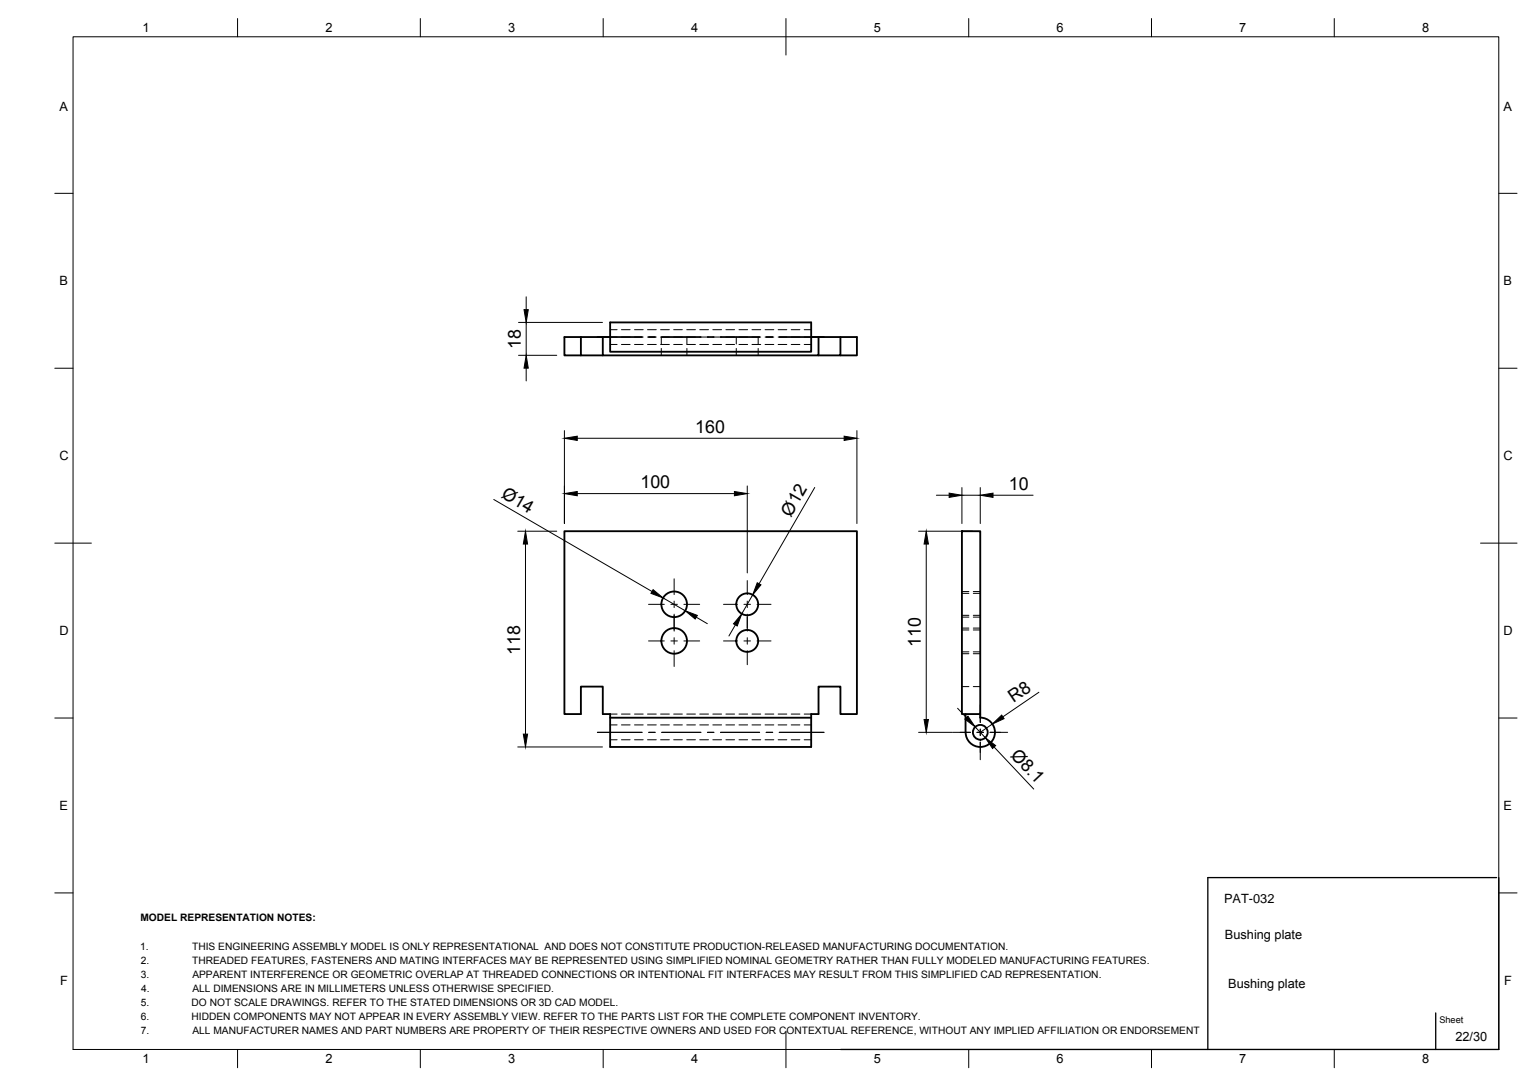
ISO-10303-21;
HEADER;
/* Generated by software containing ST-Developer
 * from STEP Tools, Inc. (www.steptools.com) 
 */

FILE_DESCRIPTION(
/* description */ ('Drill jig with bushing plate'),
/* implementation_level */ '2;1');

FILE_NAME(
/* name */ 'Bushing plate.step',
/* time_stamp */ '2026-10-27T10:51:08-07:00',
/* author */ (''),
/* organization */ (''),
/* preprocessor_version */ 'ST-DEVELOPER v20.2',
/* originating_system */ 'Autodesk Translation Framework v15.17.0.0',
/* authorisation */ '');

FILE_SCHEMA (('AUTOMOTIVE_DESIGN { 1 0 10303 214 3 1 1 }'));
ENDSEC;

DATA;
#10=MECHANICAL_DESIGN_GEOMETRIC_PRESENTATION_REPRESENTATION('',(#240),#6638);
#192=SHAPE_REPRESENTATION_RELATIONSHIP('SRR','None',#6757,#216);
#216=ADVANCED_BREP_SHAPE_REPRESENTATION('',(#262),#6630);
#240=STYLED_ITEM('',(#6957),#262);
#262=MANIFOLD_SOLID_BREP('Body1',#3609);
#345=FACE_BOUND('',#951,.T.);
#346=FACE_BOUND('',#954,.T.);
#347=FACE_BOUND('',#962,.T.);
#348=FACE_BOUND('',#963,.T.);
#349=FACE_BOUND('',#964,.T.);
#350=FACE_BOUND('',#965,.T.);
#351=FACE_BOUND('',#975,.T.);
#352=FACE_BOUND('',#976,.T.);
#353=FACE_BOUND('',#977,.T.);
#354=FACE_BOUND('',#978,.T.);
#464=PLANE('',#4221);
#465=PLANE('',#4224);
#466=PLANE('',#4225);
#467=PLANE('',#4230);
#468=PLANE('',#4231);
#469=PLANE('',#4232);
#470=PLANE('',#4233);
#471=PLANE('',#4234);
#472=PLANE('',#4235);
#473=PLANE('',#4236);
#474=PLANE('',#4237);
#475=PLANE('',#4238);
#476=PLANE('',#4239);
#477=PLANE('',#4240);
#478=PLANE('',#4241);
#479=PLANE('',#4242);
#480=PLANE('',#4243);
#656=FACE_OUTER_BOUND('',#946,.T.);
#657=FACE_OUTER_BOUND('',#947,.T.);
#658=FACE_OUTER_BOUND('',#948,.T.);
#659=FACE_OUTER_BOUND('',#949,.T.);
#660=FACE_OUTER_BOUND('',#950,.T.);
#661=FACE_OUTER_BOUND('',#952,.T.);
#662=FACE_OUTER_BOUND('',#953,.T.);
#663=FACE_OUTER_BOUND('',#955,.T.);
#664=FACE_OUTER_BOUND('',#956,.T.);
#665=FACE_OUTER_BOUND('',#957,.T.);
#666=FACE_OUTER_BOUND('',#958,.T.);
#667=FACE_OUTER_BOUND('',#959,.T.);
#668=FACE_OUTER_BOUND('',#960,.T.);
#669=FACE_OUTER_BOUND('',#961,.T.);
#670=FACE_OUTER_BOUND('',#966,.T.);
#671=FACE_OUTER_BOUND('',#967,.T.);
#672=FACE_OUTER_BOUND('',#968,.T.);
#673=FACE_OUTER_BOUND('',#969,.T.);
#674=FACE_OUTER_BOUND('',#970,.T.);
#675=FACE_OUTER_BOUND('',#971,.T.);
#676=FACE_OUTER_BOUND('',#972,.T.);
#677=FACE_OUTER_BOUND('',#973,.T.);
#678=FACE_OUTER_BOUND('',#974,.T.);
#946=EDGE_LOOP('',(#3059,#3060,#3061,#3062));
#947=EDGE_LOOP('',(#3063,#3064,#3065,#3066));
#948=EDGE_LOOP('',(#3067,#3068,#3069,#3070));
#949=EDGE_LOOP('',(#3071,#3072,#3073,#3074));
#950=EDGE_LOOP('',(#3075,#3076,#3077,#3078));
#951=EDGE_LOOP('',(#3079));
#952=EDGE_LOOP('',(#3080,#3081,#3082,#3083));
#953=EDGE_LOOP('',(#3084,#3085,#3086,#3087));
#954=EDGE_LOOP('',(#3088));
#955=EDGE_LOOP('',(#3089,#3090,#3091,#3092));
#956=EDGE_LOOP('',(#3093,#3094,#3095,#3096));
#957=EDGE_LOOP('',(#3097,#3098,#3099,#3100,#3101,#3102,#3103,#3104));
#958=EDGE_LOOP('',(#3105,#3106,#3107,#3108));
#959=EDGE_LOOP('',(#3109,#3110,#3111,#3112));
#960=EDGE_LOOP('',(#3113,#3114,#3115,#3116));
#961=EDGE_LOOP('',(#3117,#3118,#3119,#3120,#3121,#3122,#3123,#3124,#3125,
#3126,#3127,#3128,#3129,#3130,#3131,#3132));
#962=EDGE_LOOP('',(#3133));
#963=EDGE_LOOP('',(#3134));
#964=EDGE_LOOP('',(#3135));
#965=EDGE_LOOP('',(#3136));
#966=EDGE_LOOP('',(#3137,#3138,#3139,#3140));
#967=EDGE_LOOP('',(#3141,#3142,#3143,#3144));
#968=EDGE_LOOP('',(#3145,#3146,#3147,#3148));
#969=EDGE_LOOP('',(#3149,#3150,#3151,#3152));
#970=EDGE_LOOP('',(#3153,#3154,#3155,#3156));
#971=EDGE_LOOP('',(#3157,#3158,#3159,#3160));
#972=EDGE_LOOP('',(#3161,#3162,#3163,#3164));
#973=EDGE_LOOP('',(#3165,#3166,#3167,#3168));
#974=EDGE_LOOP('',(#3169,#3170,#3171,#3172,#3173,#3174,#3175,#3176,#3177,
#3178,#3179,#3180));
#975=EDGE_LOOP('',(#3181));
#976=EDGE_LOOP('',(#3182));
#977=EDGE_LOOP('',(#3183));
#978=EDGE_LOOP('',(#3184));
#1215=LINE('',#6309,#1476);
#1216=LINE('',#6315,#1477);
#1217=LINE('',#6321,#1478);
#1218=LINE('',#6327,#1479);
#1219=LINE('',#6334,#1480);
#1220=LINE('',#6336,#1481);
#1221=LINE('',#6337,#1482);
#1222=LINE('',#6342,#1483);
#1223=LINE('',#6344,#1484);
#1224=LINE('',#6345,#1485);
#1225=LINE('',#6350,#1486);
#1226=LINE('',#6351,#1487);
#1227=LINE('',#6355,#1488);
#1228=LINE('',#6357,#1489);
#1229=LINE('',#6360,#1490);
#1230=LINE('',#6362,#1491);
#1231=LINE('',#6364,#1492);
#1232=LINE('',#6366,#1493);
#1233=LINE('',#6367,#1494);
#1234=LINE('',#6370,#1495);
#1235=LINE('',#6372,#1496);
#1236=LINE('',#6373,#1497);
#1237=LINE('',#6376,#1498);
#1238=LINE('',#6378,#1499);
#1239=LINE('',#6379,#1500);
#1240=LINE('',#6382,#1501);
#1241=LINE('',#6384,#1502);
#1242=LINE('',#6385,#1503);
#1243=LINE('',#6388,#1504);
#1244=LINE('',#6390,#1505);
#1245=LINE('',#6392,#1506);
#1246=LINE('',#6394,#1507);
#1247=LINE('',#6396,#1508);
#1248=LINE('',#6398,#1509);
#1249=LINE('',#6400,#1510);
#1250=LINE('',#6401,#1511);
#1251=LINE('',#6404,#1512);
#1252=LINE('',#6405,#1513);
#1253=LINE('',#6408,#1514);
#1254=LINE('',#6409,#1515);
#1255=LINE('',#6412,#1516);
#1256=LINE('',#6413,#1517);
#1257=LINE('',#6416,#1518);
#1258=LINE('',#6417,#1519);
#1259=LINE('',#6420,#1520);
#1260=LINE('',#6421,#1521);
#1261=LINE('',#6424,#1522);
#1262=LINE('',#6426,#1523);
#1263=LINE('',#6427,#1524);
#1264=LINE('',#6429,#1525);
#1265=LINE('',#6431,#1526);
#1476=VECTOR('',#5174,0.7);
#1477=VECTOR('',#5181,0.7);
#1478=VECTOR('',#5188,0.6);
#1479=VECTOR('',#5195,0.6);
#1480=VECTOR('',#5202,1.);
#1481=VECTOR('',#5203,1.);
#1482=VECTOR('',#5204,1.);
#1483=VECTOR('',#5209,1.);
#1484=VECTOR('',#5210,1.);
#1485=VECTOR('',#5211,1.);
#1486=VECTOR('',#5216,1.);
#1487=VECTOR('',#5217,1.);
#1488=VECTOR('',#5222,0.405);
#1489=VECTOR('',#5225,1.);
#1490=VECTOR('',#5228,1.);
#1491=VECTOR('',#5229,1.);
#1492=VECTOR('',#5230,1.);
#1493=VECTOR('',#5231,1.);
#1494=VECTOR('',#5232,1.);
#1495=VECTOR('',#5235,1.);
#1496=VECTOR('',#5236,1.);
#1497=VECTOR('',#5237,1.);
#1498=VECTOR('',#5240,1.);
#1499=VECTOR('',#5241,1.);
#1500=VECTOR('',#5242,1.);
#1501=VECTOR('',#5245,1.);
#1502=VECTOR('',#5246,1.);
#1503=VECTOR('',#5247,1.);
#1504=VECTOR('',#5250,1.);
#1505=VECTOR('',#5251,1.);
#1506=VECTOR('',#5252,1.);
#1507=VECTOR('',#5253,1.);
#1508=VECTOR('',#5254,1.);
#1509=VECTOR('',#5255,1.);
#1510=VECTOR('',#5256,1.);
#1511=VECTOR('',#5257,1.);
#1512=VECTOR('',#5260,1.);
#1513=VECTOR('',#5261,1.);
#1514=VECTOR('',#5264,1.);
#1515=VECTOR('',#5265,1.);
#1516=VECTOR('',#5268,1.);
#1517=VECTOR('',#5269,1.);
#1518=VECTOR('',#5272,1.);
#1519=VECTOR('',#5273,1.);
#1520=VECTOR('',#5276,1.);
#1521=VECTOR('',#5277,1.);
#1522=VECTOR('',#5280,1.);
#1523=VECTOR('',#5281,1.);
#1524=VECTOR('',#5282,1.);
#1525=VECTOR('',#5285,1.);
#1526=VECTOR('',#5288,1.);
#1676=CIRCLE('',#4210,0.7);
#1677=CIRCLE('',#4211,0.7);
#1678=CIRCLE('',#4213,0.7);
#1679=CIRCLE('',#4214,0.7);
#1680=CIRCLE('',#4216,0.6);
#1681=CIRCLE('',#4217,0.6);
#1682=CIRCLE('',#4219,0.6);
#1683=CIRCLE('',#4220,0.6);
#1684=CIRCLE('',#4222,0.8);
#1685=CIRCLE('',#4223,0.405);
#1686=CIRCLE('',#4226,0.8);
#1687=CIRCLE('',#4227,0.405);
#1926=VERTEX_POINT('',#6306);
#1927=VERTEX_POINT('',#6308);
#1928=VERTEX_POINT('',#6312);
#1929=VERTEX_POINT('',#6314);
#1930=VERTEX_POINT('',#6318);
#1931=VERTEX_POINT('',#6320);
#1932=VERTEX_POINT('',#6324);
#1933=VERTEX_POINT('',#6326);
#1934=VERTEX_POINT('',#6330);
#1935=VERTEX_POINT('',#6331);
#1936=VERTEX_POINT('',#6333);
#1937=VERTEX_POINT('',#6335);
#1938=VERTEX_POINT('',#6338);
#1939=VERTEX_POINT('',#6341);
#1940=VERTEX_POINT('',#6343);
#1941=VERTEX_POINT('',#6347);
#1942=VERTEX_POINT('',#6349);
#1943=VERTEX_POINT('',#6352);
#1944=VERTEX_POINT('',#6359);
#1945=VERTEX_POINT('',#6361);
#1946=VERTEX_POINT('',#6363);
#1947=VERTEX_POINT('',#6365);
#1948=VERTEX_POINT('',#6369);
#1949=VERTEX_POINT('',#6371);
#1950=VERTEX_POINT('',#6375);
#1951=VERTEX_POINT('',#6377);
#1952=VERTEX_POINT('',#6381);
#1953=VERTEX_POINT('',#6383);
#1954=VERTEX_POINT('',#6387);
#1955=VERTEX_POINT('',#6389);
#1956=VERTEX_POINT('',#6391);
#1957=VERTEX_POINT('',#6393);
#1958=VERTEX_POINT('',#6395);
#1959=VERTEX_POINT('',#6397);
#1960=VERTEX_POINT('',#6399);
#1961=VERTEX_POINT('',#6403);
#1962=VERTEX_POINT('',#6407);
#1963=VERTEX_POINT('',#6411);
#1964=VERTEX_POINT('',#6415);
#1965=VERTEX_POINT('',#6419);
#1966=VERTEX_POINT('',#6423);
#1967=VERTEX_POINT('',#6425);
#2317=EDGE_CURVE('',#1926,#1926,#1676,.T.);
#2318=EDGE_CURVE('',#1926,#1927,#1215,.T.);
#2319=EDGE_CURVE('',#1927,#1927,#1677,.T.);
#2320=EDGE_CURVE('',#1928,#1928,#1678,.T.);
#2321=EDGE_CURVE('',#1928,#1929,#1216,.T.);
#2322=EDGE_CURVE('',#1929,#1929,#1679,.T.);
#2323=EDGE_CURVE('',#1930,#1930,#1680,.T.);
#2324=EDGE_CURVE('',#1930,#1931,#1217,.T.);
#2325=EDGE_CURVE('',#1931,#1931,#1681,.T.);
#2326=EDGE_CURVE('',#1932,#1932,#1682,.T.);
#2327=EDGE_CURVE('',#1932,#1933,#1218,.T.);
#2328=EDGE_CURVE('',#1933,#1933,#1683,.T.);
#2329=EDGE_CURVE('',#1934,#1935,#1684,.T.);
#2330=EDGE_CURVE('',#1936,#1934,#1219,.T.);
#2331=EDGE_CURVE('',#1937,#1936,#1220,.T.);
#2332=EDGE_CURVE('',#1935,#1937,#1221,.T.);
#2333=EDGE_CURVE('',#1938,#1938,#1685,.T.);
#2334=EDGE_CURVE('',#1936,#1939,#1222,.T.);
#2335=EDGE_CURVE('',#1934,#1940,#1223,.T.);
#2336=EDGE_CURVE('',#1939,#1940,#1224,.T.);
#2337=EDGE_CURVE('',#1940,#1941,#1686,.T.);
#2338=EDGE_CURVE('',#1941,#1942,#1225,.T.);
#2339=EDGE_CURVE('',#1939,#1942,#1226,.T.);
#2340=EDGE_CURVE('',#1943,#1943,#1687,.T.);
#2341=EDGE_CURVE('',#1943,#1938,#1227,.T.);
#2342=EDGE_CURVE('',#1935,#1941,#1228,.T.);
#2343=EDGE_CURVE('',#1942,#1944,#1229,.T.);
#2344=EDGE_CURVE('',#1944,#1945,#1230,.T.);
#2345=EDGE_CURVE('',#1946,#1945,#1231,.T.);
#2346=EDGE_CURVE('',#1946,#1947,#1232,.T.);
#2347=EDGE_CURVE('',#1947,#1937,#1233,.T.);
#2348=EDGE_CURVE('',#1948,#1944,#1234,.T.);
#2349=EDGE_CURVE('',#1948,#1949,#1235,.T.);
#2350=EDGE_CURVE('',#1945,#1949,#1236,.T.);
#2351=EDGE_CURVE('',#1950,#1948,#1237,.T.);
#2352=EDGE_CURVE('',#1950,#1951,#1238,.T.);
#2353=EDGE_CURVE('',#1949,#1951,#1239,.T.);
#2354=EDGE_CURVE('',#1952,#1950,#1240,.T.);
#2355=EDGE_CURVE('',#1953,#1952,#1241,.T.);
#2356=EDGE_CURVE('',#1951,#1953,#1242,.T.);
#2357=EDGE_CURVE('',#1947,#1954,#1243,.T.);
#2358=EDGE_CURVE('',#1954,#1955,#1244,.T.);
#2359=EDGE_CURVE('',#1955,#1956,#1245,.T.);
#2360=EDGE_CURVE('',#1957,#1956,#1246,.T.);
#2361=EDGE_CURVE('',#1958,#1957,#1247,.T.);
#2362=EDGE_CURVE('',#1959,#1958,#1248,.T.);
#2363=EDGE_CURVE('',#1960,#1959,#1249,.T.);
#2364=EDGE_CURVE('',#1952,#1960,#1250,.T.);
#2365=EDGE_CURVE('',#1961,#1946,#1251,.T.);
#2366=EDGE_CURVE('',#1954,#1961,#1252,.T.);
#2367=EDGE_CURVE('',#1962,#1961,#1253,.T.);
#2368=EDGE_CURVE('',#1955,#1962,#1254,.T.);
#2369=EDGE_CURVE('',#1963,#1962,#1255,.T.);
#2370=EDGE_CURVE('',#1956,#1963,#1256,.T.);
#2371=EDGE_CURVE('',#1964,#1963,#1257,.T.);
#2372=EDGE_CURVE('',#1957,#1964,#1258,.T.);
#2373=EDGE_CURVE('',#1960,#1965,#1259,.T.);
#2374=EDGE_CURVE('',#1953,#1965,#1260,.T.);
#2375=EDGE_CURVE('',#1958,#1966,#1261,.T.);
#2376=EDGE_CURVE('',#1967,#1966,#1262,.T.);
#2377=EDGE_CURVE('',#1959,#1967,#1263,.T.);
#2378=EDGE_CURVE('',#1965,#1967,#1264,.T.);
#2379=EDGE_CURVE('',#1966,#1964,#1265,.T.);
#3059=ORIENTED_EDGE('',*,*,#2317,.F.);
#3060=ORIENTED_EDGE('',*,*,#2318,.T.);
#3061=ORIENTED_EDGE('',*,*,#2319,.F.);
#3062=ORIENTED_EDGE('',*,*,#2318,.F.);
#3063=ORIENTED_EDGE('',*,*,#2320,.F.);
#3064=ORIENTED_EDGE('',*,*,#2321,.T.);
#3065=ORIENTED_EDGE('',*,*,#2322,.F.);
#3066=ORIENTED_EDGE('',*,*,#2321,.F.);
#3067=ORIENTED_EDGE('',*,*,#2323,.F.);
#3068=ORIENTED_EDGE('',*,*,#2324,.T.);
#3069=ORIENTED_EDGE('',*,*,#2325,.F.);
#3070=ORIENTED_EDGE('',*,*,#2324,.F.);
#3071=ORIENTED_EDGE('',*,*,#2326,.F.);
#3072=ORIENTED_EDGE('',*,*,#2327,.T.);
#3073=ORIENTED_EDGE('',*,*,#2328,.F.);
#3074=ORIENTED_EDGE('',*,*,#2327,.F.);
#3075=ORIENTED_EDGE('',*,*,#2329,.F.);
#3076=ORIENTED_EDGE('',*,*,#2330,.F.);
#3077=ORIENTED_EDGE('',*,*,#2331,.F.);
#3078=ORIENTED_EDGE('',*,*,#2332,.F.);
#3079=ORIENTED_EDGE('',*,*,#2333,.F.);
#3080=ORIENTED_EDGE('',*,*,#2334,.F.);
#3081=ORIENTED_EDGE('',*,*,#2330,.T.);
#3082=ORIENTED_EDGE('',*,*,#2335,.T.);
#3083=ORIENTED_EDGE('',*,*,#2336,.F.);
#3084=ORIENTED_EDGE('',*,*,#2337,.T.);
#3085=ORIENTED_EDGE('',*,*,#2338,.T.);
#3086=ORIENTED_EDGE('',*,*,#2339,.F.);
#3087=ORIENTED_EDGE('',*,*,#2336,.T.);
#3088=ORIENTED_EDGE('',*,*,#2340,.T.);
#3089=ORIENTED_EDGE('',*,*,#2340,.F.);
#3090=ORIENTED_EDGE('',*,*,#2341,.T.);
#3091=ORIENTED_EDGE('',*,*,#2333,.T.);
#3092=ORIENTED_EDGE('',*,*,#2341,.F.);
#3093=ORIENTED_EDGE('',*,*,#2342,.T.);
#3094=ORIENTED_EDGE('',*,*,#2337,.F.);
#3095=ORIENTED_EDGE('',*,*,#2335,.F.);
#3096=ORIENTED_EDGE('',*,*,#2329,.T.);
#3097=ORIENTED_EDGE('',*,*,#2331,.T.);
#3098=ORIENTED_EDGE('',*,*,#2334,.T.);
#3099=ORIENTED_EDGE('',*,*,#2339,.T.);
#3100=ORIENTED_EDGE('',*,*,#2343,.T.);
#3101=ORIENTED_EDGE('',*,*,#2344,.T.);
#3102=ORIENTED_EDGE('',*,*,#2345,.F.);
#3103=ORIENTED_EDGE('',*,*,#2346,.T.);
#3104=ORIENTED_EDGE('',*,*,#2347,.T.);
#3105=ORIENTED_EDGE('',*,*,#2348,.F.);
#3106=ORIENTED_EDGE('',*,*,#2349,.T.);
#3107=ORIENTED_EDGE('',*,*,#2350,.F.);
#3108=ORIENTED_EDGE('',*,*,#2344,.F.);
#3109=ORIENTED_EDGE('',*,*,#2351,.F.);
#3110=ORIENTED_EDGE('',*,*,#2352,.T.);
#3111=ORIENTED_EDGE('',*,*,#2353,.F.);
#3112=ORIENTED_EDGE('',*,*,#2349,.F.);
#3113=ORIENTED_EDGE('',*,*,#2354,.F.);
#3114=ORIENTED_EDGE('',*,*,#2355,.F.);
#3115=ORIENTED_EDGE('',*,*,#2356,.F.);
#3116=ORIENTED_EDGE('',*,*,#2352,.F.);
#3117=ORIENTED_EDGE('',*,*,#2347,.F.);
#3118=ORIENTED_EDGE('',*,*,#2357,.T.);
#3119=ORIENTED_EDGE('',*,*,#2358,.T.);
#3120=ORIENTED_EDGE('',*,*,#2359,.T.);
#3121=ORIENTED_EDGE('',*,*,#2360,.F.);
#3122=ORIENTED_EDGE('',*,*,#2361,.F.);
#3123=ORIENTED_EDGE('',*,*,#2362,.F.);
#3124=ORIENTED_EDGE('',*,*,#2363,.F.);
#3125=ORIENTED_EDGE('',*,*,#2364,.F.);
#3126=ORIENTED_EDGE('',*,*,#2354,.T.);
#3127=ORIENTED_EDGE('',*,*,#2351,.T.);
#3128=ORIENTED_EDGE('',*,*,#2348,.T.);
#3129=ORIENTED_EDGE('',*,*,#2343,.F.);
#3130=ORIENTED_EDGE('',*,*,#2338,.F.);
#3131=ORIENTED_EDGE('',*,*,#2342,.F.);
#3132=ORIENTED_EDGE('',*,*,#2332,.T.);
#3133=ORIENTED_EDGE('',*,*,#2317,.T.);
#3134=ORIENTED_EDGE('',*,*,#2320,.T.);
#3135=ORIENTED_EDGE('',*,*,#2323,.T.);
#3136=ORIENTED_EDGE('',*,*,#2326,.T.);
#3137=ORIENTED_EDGE('',*,*,#2365,.F.);
#3138=ORIENTED_EDGE('',*,*,#2366,.F.);
#3139=ORIENTED_EDGE('',*,*,#2357,.F.);
#3140=ORIENTED_EDGE('',*,*,#2346,.F.);
#3141=ORIENTED_EDGE('',*,*,#2367,.F.);
#3142=ORIENTED_EDGE('',*,*,#2368,.F.);
#3143=ORIENTED_EDGE('',*,*,#2358,.F.);
#3144=ORIENTED_EDGE('',*,*,#2366,.T.);
#3145=ORIENTED_EDGE('',*,*,#2369,.F.);
#3146=ORIENTED_EDGE('',*,*,#2370,.F.);
#3147=ORIENTED_EDGE('',*,*,#2359,.F.);
#3148=ORIENTED_EDGE('',*,*,#2368,.T.);
#3149=ORIENTED_EDGE('',*,*,#2370,.T.);
#3150=ORIENTED_EDGE('',*,*,#2371,.F.);
#3151=ORIENTED_EDGE('',*,*,#2372,.F.);
#3152=ORIENTED_EDGE('',*,*,#2360,.T.);
#3153=ORIENTED_EDGE('',*,*,#2355,.T.);
#3154=ORIENTED_EDGE('',*,*,#2364,.T.);
#3155=ORIENTED_EDGE('',*,*,#2373,.T.);
#3156=ORIENTED_EDGE('',*,*,#2374,.F.);
#3157=ORIENTED_EDGE('',*,*,#2362,.T.);
#3158=ORIENTED_EDGE('',*,*,#2375,.T.);
#3159=ORIENTED_EDGE('',*,*,#2376,.F.);
#3160=ORIENTED_EDGE('',*,*,#2377,.F.);
#3161=ORIENTED_EDGE('',*,*,#2363,.T.);
#3162=ORIENTED_EDGE('',*,*,#2377,.T.);
#3163=ORIENTED_EDGE('',*,*,#2378,.F.);
#3164=ORIENTED_EDGE('',*,*,#2373,.F.);
#3165=ORIENTED_EDGE('',*,*,#2361,.T.);
#3166=ORIENTED_EDGE('',*,*,#2372,.T.);
#3167=ORIENTED_EDGE('',*,*,#2379,.F.);
#3168=ORIENTED_EDGE('',*,*,#2375,.F.);
#3169=ORIENTED_EDGE('',*,*,#2356,.T.);
#3170=ORIENTED_EDGE('',*,*,#2374,.T.);
#3171=ORIENTED_EDGE('',*,*,#2378,.T.);
#3172=ORIENTED_EDGE('',*,*,#2376,.T.);
#3173=ORIENTED_EDGE('',*,*,#2379,.T.);
#3174=ORIENTED_EDGE('',*,*,#2371,.T.);
#3175=ORIENTED_EDGE('',*,*,#2369,.T.);
#3176=ORIENTED_EDGE('',*,*,#2367,.T.);
#3177=ORIENTED_EDGE('',*,*,#2365,.T.);
#3178=ORIENTED_EDGE('',*,*,#2345,.T.);
#3179=ORIENTED_EDGE('',*,*,#2350,.T.);
#3180=ORIENTED_EDGE('',*,*,#2353,.T.);
#3181=ORIENTED_EDGE('',*,*,#2319,.T.);
#3182=ORIENTED_EDGE('',*,*,#2322,.T.);
#3183=ORIENTED_EDGE('',*,*,#2325,.T.);
#3184=ORIENTED_EDGE('',*,*,#2328,.T.);
#3354=CYLINDRICAL_SURFACE('',#4209,0.7);
#3355=CYLINDRICAL_SURFACE('',#4212,0.7);
#3356=CYLINDRICAL_SURFACE('',#4215,0.6);
#3357=CYLINDRICAL_SURFACE('',#4218,0.6);
#3358=CYLINDRICAL_SURFACE('',#4228,0.405);
#3359=CYLINDRICAL_SURFACE('',#4229,0.8);
#3531=ADVANCED_FACE('',(#656),#3354,.F.);
#3532=ADVANCED_FACE('',(#657),#3355,.F.);
#3533=ADVANCED_FACE('',(#658),#3356,.F.);
#3534=ADVANCED_FACE('',(#659),#3357,.F.);
#3535=ADVANCED_FACE('',(#660,#345),#464,.F.);
#3536=ADVANCED_FACE('',(#661),#465,.T.);
#3537=ADVANCED_FACE('',(#662,#346),#466,.T.);
#3538=ADVANCED_FACE('',(#663),#3358,.F.);
#3539=ADVANCED_FACE('',(#664),#3359,.T.);
#3540=ADVANCED_FACE('',(#665),#467,.T.);
#3541=ADVANCED_FACE('',(#666),#468,.F.);
#3542=ADVANCED_FACE('',(#667),#469,.F.);
#3543=ADVANCED_FACE('',(#668),#470,.F.);
#3544=ADVANCED_FACE('',(#669,#347,#348,#349,#350),#471,.F.);
#3545=ADVANCED_FACE('',(#670),#472,.F.);
#3546=ADVANCED_FACE('',(#671),#473,.F.);
#3547=ADVANCED_FACE('',(#672),#474,.F.);
#3548=ADVANCED_FACE('',(#673),#475,.T.);
#3549=ADVANCED_FACE('',(#674),#476,.T.);
#3550=ADVANCED_FACE('',(#675),#477,.T.);
#3551=ADVANCED_FACE('',(#676),#478,.T.);
#3552=ADVANCED_FACE('',(#677),#479,.T.);
#3553=ADVANCED_FACE('',(#678,#351,#352,#353,#354),#480,.T.);
#3609=CLOSED_SHELL('',(#3531,#3532,#3533,#3534,#3535,#3536,#3537,#3538,
#3539,#3540,#3541,#3542,#3543,#3544,#3545,#3546,#3547,#3548,#3549,#3550,
#3551,#3552,#3553));
#4208=AXIS2_PLACEMENT_3D('',#6304,#5168,#5169);
#4209=AXIS2_PLACEMENT_3D('',#6305,#5170,#5171);
#4210=AXIS2_PLACEMENT_3D('',#6307,#5172,#5173);
#4211=AXIS2_PLACEMENT_3D('',#6310,#5175,#5176);
#4212=AXIS2_PLACEMENT_3D('',#6311,#5177,#5178);
#4213=AXIS2_PLACEMENT_3D('',#6313,#5179,#5180);
#4214=AXIS2_PLACEMENT_3D('',#6316,#5182,#5183);
#4215=AXIS2_PLACEMENT_3D('',#6317,#5184,#5185);
#4216=AXIS2_PLACEMENT_3D('',#6319,#5186,#5187);
#4217=AXIS2_PLACEMENT_3D('',#6322,#5189,#5190);
#4218=AXIS2_PLACEMENT_3D('',#6323,#5191,#5192);
#4219=AXIS2_PLACEMENT_3D('',#6325,#5193,#5194);
#4220=AXIS2_PLACEMENT_3D('',#6328,#5196,#5197);
#4221=AXIS2_PLACEMENT_3D('',#6329,#5198,#5199);
#4222=AXIS2_PLACEMENT_3D('',#6332,#5200,#5201);
#4223=AXIS2_PLACEMENT_3D('',#6339,#5205,#5206);
#4224=AXIS2_PLACEMENT_3D('',#6340,#5207,#5208);
#4225=AXIS2_PLACEMENT_3D('',#6346,#5212,#5213);
#4226=AXIS2_PLACEMENT_3D('',#6348,#5214,#5215);
#4227=AXIS2_PLACEMENT_3D('',#6353,#5218,#5219);
#4228=AXIS2_PLACEMENT_3D('',#6354,#5220,#5221);
#4229=AXIS2_PLACEMENT_3D('',#6356,#5223,#5224);
#4230=AXIS2_PLACEMENT_3D('',#6358,#5226,#5227);
#4231=AXIS2_PLACEMENT_3D('',#6368,#5233,#5234);
#4232=AXIS2_PLACEMENT_3D('',#6374,#5238,#5239);
#4233=AXIS2_PLACEMENT_3D('',#6380,#5243,#5244);
#4234=AXIS2_PLACEMENT_3D('',#6386,#5248,#5249);
#4235=AXIS2_PLACEMENT_3D('',#6402,#5258,#5259);
#4236=AXIS2_PLACEMENT_3D('',#6406,#5262,#5263);
#4237=AXIS2_PLACEMENT_3D('',#6410,#5266,#5267);
#4238=AXIS2_PLACEMENT_3D('',#6414,#5270,#5271);
#4239=AXIS2_PLACEMENT_3D('',#6418,#5274,#5275);
#4240=AXIS2_PLACEMENT_3D('',#6422,#5278,#5279);
#4241=AXIS2_PLACEMENT_3D('',#6428,#5283,#5284);
#4242=AXIS2_PLACEMENT_3D('',#6430,#5286,#5287);
#4243=AXIS2_PLACEMENT_3D('',#6432,#5289,#5290);
#5168=DIRECTION('axis',(0.,0.,1.));
#5169=DIRECTION('refdir',(1.,0.,0.));
#5170=DIRECTION('center_axis',(0.,0.,1.));
#5171=DIRECTION('ref_axis',(1.,0.,0.));
#5172=DIRECTION('center_axis',(0.,0.,1.));
#5173=DIRECTION('ref_axis',(1.,0.,0.));
#5174=DIRECTION('',(0.,0.,1.));
#5175=DIRECTION('center_axis',(0.,0.,-1.));
#5176=DIRECTION('ref_axis',(1.,0.,0.));
#5177=DIRECTION('center_axis',(0.,0.,1.));
#5178=DIRECTION('ref_axis',(1.,0.,0.));
#5179=DIRECTION('center_axis',(0.,0.,1.));
#5180=DIRECTION('ref_axis',(1.,0.,0.));
#5181=DIRECTION('',(0.,0.,1.));
#5182=DIRECTION('center_axis',(0.,0.,-1.));
#5183=DIRECTION('ref_axis',(1.,0.,0.));
#5184=DIRECTION('center_axis',(0.,0.,1.));
#5185=DIRECTION('ref_axis',(1.,0.,0.));
#5186=DIRECTION('center_axis',(0.,0.,1.));
#5187=DIRECTION('ref_axis',(1.,0.,0.));
#5188=DIRECTION('',(0.,0.,1.));
#5189=DIRECTION('center_axis',(0.,0.,-1.));
#5190=DIRECTION('ref_axis',(1.,0.,0.));
#5191=DIRECTION('center_axis',(0.,0.,1.));
#5192=DIRECTION('ref_axis',(1.,0.,0.));
#5193=DIRECTION('center_axis',(0.,0.,1.));
#5194=DIRECTION('ref_axis',(1.,0.,0.));
#5195=DIRECTION('',(0.,0.,1.));
#5196=DIRECTION('center_axis',(0.,0.,-1.));
#5197=DIRECTION('ref_axis',(1.,0.,0.));
#5198=DIRECTION('center_axis',(1.,0.,0.));
#5199=DIRECTION('ref_axis',(0.,0.,-1.));
#5200=DIRECTION('center_axis',(1.,0.,0.));
#5201=DIRECTION('ref_axis',(0.,0.,-1.));
#5202=DIRECTION('',(0.,-1.,0.));
#5203=DIRECTION('',(0.,0.,1.));
#5204=DIRECTION('',(0.,1.,0.));
#5205=DIRECTION('center_axis',(-1.,0.,0.));
#5206=DIRECTION('ref_axis',(0.,0.,-1.));
#5207=DIRECTION('center_axis',(0.,0.,1.));
#5208=DIRECTION('ref_axis',(0.,-1.,0.));
#5209=DIRECTION('',(1.,0.,0.));
#5210=DIRECTION('',(1.,0.,0.));
#5211=DIRECTION('',(0.,-1.,0.));
#5212=DIRECTION('center_axis',(1.,0.,0.));
#5213=DIRECTION('ref_axis',(0.,0.,-1.));
#5214=DIRECTION('center_axis',(1.,0.,0.));
#5215=DIRECTION('ref_axis',(0.,0.,-1.));
#5216=DIRECTION('',(0.,1.,0.));
#5217=DIRECTION('',(0.,0.,-1.));
#5218=DIRECTION('center_axis',(-1.,0.,0.));
#5219=DIRECTION('ref_axis',(0.,0.,-1.));
#5220=DIRECTION('center_axis',(1.,0.,0.));
#5221=DIRECTION('ref_axis',(0.,0.,-1.));
#5222=DIRECTION('',(-1.,0.,0.));
#5223=DIRECTION('center_axis',(1.,0.,0.));
#5224=DIRECTION('ref_axis',(0.,0.,-1.));
#5225=DIRECTION('',(1.,0.,0.));
#5226=DIRECTION('center_axis',(0.,-1.,0.));
#5227=DIRECTION('ref_axis',(1.,0.,0.));
#5228=DIRECTION('',(1.,0.,0.));
#5229=DIRECTION('',(0.,0.,1.));
#5230=DIRECTION('',(1.,0.,0.));
#5231=DIRECTION('',(0.,0.,-1.));
#5232=DIRECTION('',(1.,0.,0.));
#5233=DIRECTION('center_axis',(-1.,0.,0.));
#5234=DIRECTION('ref_axis',(0.,-1.,0.));
#5235=DIRECTION('',(0.,-1.,0.));
#5236=DIRECTION('',(0.,0.,1.));
#5237=DIRECTION('',(0.,1.,0.));
#5238=DIRECTION('center_axis',(0.,1.,0.));
#5239=DIRECTION('ref_axis',(-1.,0.,0.));
#5240=DIRECTION('',(-1.,0.,0.));
#5241=DIRECTION('',(0.,0.,1.));
#5242=DIRECTION('',(1.,0.,0.));
#5243=DIRECTION('center_axis',(1.,0.,0.));
#5244=DIRECTION('ref_axis',(0.,1.,0.));
#5245=DIRECTION('',(0.,1.,0.));
#5246=DIRECTION('',(0.,0.,-1.));
#5247=DIRECTION('',(0.,-1.,0.));
#5248=DIRECTION('center_axis',(0.,0.,1.));
#5249=DIRECTION('ref_axis',(1.,0.,0.));
#5250=DIRECTION('',(0.,1.,0.));
#5251=DIRECTION('',(-1.,0.,0.));
#5252=DIRECTION('',(0.,-1.,0.));
#5253=DIRECTION('',(1.,0.,0.));
#5254=DIRECTION('',(0.,-1.,0.));
#5255=DIRECTION('',(-1.,0.,0.));
#5256=DIRECTION('',(0.,1.,0.));
#5257=DIRECTION('',(1.,0.,0.));
#5258=DIRECTION('center_axis',(1.,0.,0.));
#5259=DIRECTION('ref_axis',(0.,1.,0.));
#5260=DIRECTION('',(0.,-1.,0.));
#5261=DIRECTION('',(0.,0.,1.));
#5262=DIRECTION('center_axis',(0.,1.,0.));
#5263=DIRECTION('ref_axis',(-1.,0.,0.));
#5264=DIRECTION('',(1.,0.,0.));
#5265=DIRECTION('',(0.,0.,1.));
#5266=DIRECTION('center_axis',(-1.,0.,0.));
#5267=DIRECTION('ref_axis',(0.,-1.,0.));
#5268=DIRECTION('',(0.,1.,0.));
#5269=DIRECTION('',(0.,0.,1.));
#5270=DIRECTION('center_axis',(0.,-1.,0.));
#5271=DIRECTION('ref_axis',(1.,0.,0.));
#5272=DIRECTION('',(1.,0.,0.));
#5273=DIRECTION('',(0.,0.,1.));
#5274=DIRECTION('center_axis',(0.,-1.,0.));
#5275=DIRECTION('ref_axis',(1.,0.,0.));
#5276=DIRECTION('',(0.,0.,1.));
#5277=DIRECTION('',(1.,0.,0.));
#5278=DIRECTION('center_axis',(0.,1.,0.));
#5279=DIRECTION('ref_axis',(-1.,0.,0.));
#5280=DIRECTION('',(0.,0.,1.));
#5281=DIRECTION('',(-1.,0.,0.));
#5282=DIRECTION('',(0.,0.,1.));
#5283=DIRECTION('center_axis',(1.,0.,0.));
#5284=DIRECTION('ref_axis',(0.,1.,0.));
#5285=DIRECTION('',(0.,1.,0.));
#5286=DIRECTION('center_axis',(-1.,0.,0.));
#5287=DIRECTION('ref_axis',(0.,-1.,0.));
#5288=DIRECTION('',(0.,-1.,0.));
#5289=DIRECTION('center_axis',(0.,0.,1.));
#5290=DIRECTION('ref_axis',(1.,0.,0.));
#6304=CARTESIAN_POINT('',(0.,0.,0.));
#6305=CARTESIAN_POINT('Origin',(2.,1.,3.4));
#6306=CARTESIAN_POINT('',(1.3,1.,3.5));
#6307=CARTESIAN_POINT('Origin',(2.,1.,3.5));
#6308=CARTESIAN_POINT('',(1.3,1.,4.5));
#6309=CARTESIAN_POINT('',(1.3,1.,3.4));
#6310=CARTESIAN_POINT('Origin',(2.,1.,4.5));
#6311=CARTESIAN_POINT('Origin',(2.,-1.,3.4));
#6312=CARTESIAN_POINT('',(1.3,-1.,3.5));
#6313=CARTESIAN_POINT('Origin',(2.,-1.,3.5));
#6314=CARTESIAN_POINT('',(1.3,-1.,4.5));
#6315=CARTESIAN_POINT('',(1.3,-1.,3.4));
#6316=CARTESIAN_POINT('Origin',(2.,-1.,4.5));
#6317=CARTESIAN_POINT('Origin',(-2.,1.,3.4));
#6318=CARTESIAN_POINT('',(-2.6,1.,3.5));
#6319=CARTESIAN_POINT('Origin',(-2.,1.,3.5));
#6320=CARTESIAN_POINT('',(-2.6,1.,4.5));
#6321=CARTESIAN_POINT('',(-2.6,1.,3.4));
#6322=CARTESIAN_POINT('Origin',(-2.,1.,4.5));
#6323=CARTESIAN_POINT('Origin',(-2.,-1.,3.4));
#6324=CARTESIAN_POINT('',(-2.6,-1.,3.5));
#6325=CARTESIAN_POINT('Origin',(-2.,-1.,3.5));
#6326=CARTESIAN_POINT('',(-2.6,-1.,4.5));
#6327=CARTESIAN_POINT('',(-2.6,-1.,3.4));
#6328=CARTESIAN_POINT('Origin',(-2.,-1.,4.5));
#6329=CARTESIAN_POINT('Origin',(-5.5,-6.,3.5));
#6330=CARTESIAN_POINT('',(-5.5,-6.,4.3));
#6331=CARTESIAN_POINT('',(-5.5,-5.2,3.5));
#6332=CARTESIAN_POINT('Origin',(-5.5,-6.,3.5));
#6333=CARTESIAN_POINT('',(-5.5,-5.,4.3));
#6334=CARTESIAN_POINT('',(-5.5,-4.5,4.3));
#6335=CARTESIAN_POINT('',(-5.5,-5.,3.5));
#6336=CARTESIAN_POINT('',(-5.5,-5.,3.7));
#6337=CARTESIAN_POINT('',(-5.5,-6.,3.5));
#6338=CARTESIAN_POINT('',(-5.5,-6.,3.905));
#6339=CARTESIAN_POINT('Origin',(-5.5,-6.,3.5));
#6340=CARTESIAN_POINT('Origin',(-5.5,-4.5,4.3));
#6341=CARTESIAN_POINT('',(5.5,-5.,4.3));
#6342=CARTESIAN_POINT('',(-6.75,-5.,4.3));
#6343=CARTESIAN_POINT('',(5.5,-6.,4.3));
#6344=CARTESIAN_POINT('',(-5.5,-6.,4.3));
#6345=CARTESIAN_POINT('',(5.5,-4.5,4.3));
#6346=CARTESIAN_POINT('Origin',(5.5,-6.,3.5));
#6347=CARTESIAN_POINT('',(5.5,-5.2,3.5));
#6348=CARTESIAN_POINT('Origin',(5.5,-6.,3.5));
#6349=CARTESIAN_POINT('',(5.5,-5.,3.5));
#6350=CARTESIAN_POINT('',(5.5,-6.,3.5));
#6351=CARTESIAN_POINT('',(5.5,-5.,3.7));
#6352=CARTESIAN_POINT('',(5.5,-6.,3.905));
#6353=CARTESIAN_POINT('Origin',(5.5,-6.,3.5));
#6354=CARTESIAN_POINT('Origin',(-5.5,-6.,3.5));
#6355=CARTESIAN_POINT('',(-5.5,-6.,3.905));
#6356=CARTESIAN_POINT('Origin',(-5.5,-6.,3.5));
#6357=CARTESIAN_POINT('',(-5.5,-5.2,3.5));
#6358=CARTESIAN_POINT('Origin',(-8.,-5.,3.5));
#6359=CARTESIAN_POINT('',(5.9,-5.,3.5));
#6360=CARTESIAN_POINT('',(-8.,-5.,3.5));
#6361=CARTESIAN_POINT('',(5.9,-5.,4.5));
#6362=CARTESIAN_POINT('',(5.9,-5.,3.45));
#6363=CARTESIAN_POINT('',(-5.9,-5.,4.5));
#6364=CARTESIAN_POINT('',(-8.,-5.,4.5));
#6365=CARTESIAN_POINT('',(-5.9,-5.,3.5));
#6366=CARTESIAN_POINT('',(-5.9,-5.,3.45));
#6367=CARTESIAN_POINT('',(-8.,-5.,3.5));
#6368=CARTESIAN_POINT('Origin',(5.9,-3.5,3.4));
#6369=CARTESIAN_POINT('',(5.9,-3.5,3.5));
#6370=CARTESIAN_POINT('',(5.9,-1.75,3.5));
#6371=CARTESIAN_POINT('',(5.9,-3.5,4.5));
#6372=CARTESIAN_POINT('',(5.9,-3.5,3.4));
#6373=CARTESIAN_POINT('',(5.9,-1.75,4.5));
#6374=CARTESIAN_POINT('Origin',(7.1,-3.5,3.4));
#6375=CARTESIAN_POINT('',(7.1,-3.5,3.5));
#6376=CARTESIAN_POINT('',(3.55,-3.5,3.5));
#6377=CARTESIAN_POINT('',(7.1,-3.5,4.5));
#6378=CARTESIAN_POINT('',(7.1,-3.5,3.4));
#6379=CARTESIAN_POINT('',(3.55,-3.5,4.5));
#6380=CARTESIAN_POINT('Origin',(7.1,-5.1,3.4));
#6381=CARTESIAN_POINT('',(7.1,-5.,3.5));
#6382=CARTESIAN_POINT('',(7.1,-2.55,3.5));
#6383=CARTESIAN_POINT('',(7.1,-5.,4.5));
#6384=CARTESIAN_POINT('',(7.1,-5.,3.45));
#6385=CARTESIAN_POINT('',(7.1,-2.55,4.5));
#6386=CARTESIAN_POINT('Origin',(0.,0.,3.5));
#6387=CARTESIAN_POINT('',(-5.9,-3.5,3.5));
#6388=CARTESIAN_POINT('',(-5.9,-2.55,3.5));
#6389=CARTESIAN_POINT('',(-7.1,-3.5,3.5));
#6390=CARTESIAN_POINT('',(-2.95,-3.5,3.5));
#6391=CARTESIAN_POINT('',(-7.1,-5.,3.5));
#6392=CARTESIAN_POINT('',(-7.1,-1.75,3.5));
#6393=CARTESIAN_POINT('',(-8.,-5.,3.5));
#6394=CARTESIAN_POINT('',(-8.,-5.,3.5));
#6395=CARTESIAN_POINT('',(-8.,5.,3.5));
#6396=CARTESIAN_POINT('',(-8.,5.,3.5));
#6397=CARTESIAN_POINT('',(8.,5.,3.5));
#6398=CARTESIAN_POINT('',(8.,5.,3.5));
#6399=CARTESIAN_POINT('',(8.,-5.,3.5));
#6400=CARTESIAN_POINT('',(8.,-5.,3.5));
#6401=CARTESIAN_POINT('',(-8.,-5.,3.5));
#6402=CARTESIAN_POINT('Origin',(-5.9,-5.1,3.4));
#6403=CARTESIAN_POINT('',(-5.9,-3.5,4.5));
#6404=CARTESIAN_POINT('',(-5.9,-2.55,4.5));
#6405=CARTESIAN_POINT('',(-5.9,-3.5,3.4));
#6406=CARTESIAN_POINT('Origin',(-5.9,-3.5,3.4));
#6407=CARTESIAN_POINT('',(-7.1,-3.5,4.5));
#6408=CARTESIAN_POINT('',(-2.95,-3.5,4.5));
#6409=CARTESIAN_POINT('',(-7.1,-3.5,3.4));
#6410=CARTESIAN_POINT('Origin',(-7.1,-3.5,3.4));
#6411=CARTESIAN_POINT('',(-7.1,-5.,4.5));
#6412=CARTESIAN_POINT('',(-7.1,-1.75,4.5));
#6413=CARTESIAN_POINT('',(-7.1,-5.,3.45));
#6414=CARTESIAN_POINT('Origin',(-8.,-5.,3.5));
#6415=CARTESIAN_POINT('',(-8.,-5.,4.5));
#6416=CARTESIAN_POINT('',(-8.,-5.,4.5));
#6417=CARTESIAN_POINT('',(-8.,-5.,3.5));
#6418=CARTESIAN_POINT('Origin',(-8.,-5.,3.5));
#6419=CARTESIAN_POINT('',(8.,-5.,4.5));
#6420=CARTESIAN_POINT('',(8.,-5.,3.5));
#6421=CARTESIAN_POINT('',(-8.,-5.,4.5));
#6422=CARTESIAN_POINT('Origin',(8.,5.,3.5));
#6423=CARTESIAN_POINT('',(-8.,5.,4.5));
#6424=CARTESIAN_POINT('',(-8.,5.,3.5));
#6425=CARTESIAN_POINT('',(8.,5.,4.5));
#6426=CARTESIAN_POINT('',(8.,5.,4.5));
#6427=CARTESIAN_POINT('',(8.,5.,3.5));
#6428=CARTESIAN_POINT('Origin',(8.,-5.,3.5));
#6429=CARTESIAN_POINT('',(8.,-5.,4.5));
#6430=CARTESIAN_POINT('Origin',(-8.,5.,3.5));
#6431=CARTESIAN_POINT('',(-8.,5.,4.5));
#6432=CARTESIAN_POINT('Origin',(0.,0.,4.5));
#6601=UNCERTAINTY_MEASURE_WITH_UNIT(LENGTH_MEASURE(0.001),#6639,
'DISTANCE_ACCURACY_VALUE',
'Maximum model space distance between geometric entities at asserted c
onnectivities');
#6609=UNCERTAINTY_MEASURE_WITH_UNIT(LENGTH_MEASURE(0.001),#6639,
'DISTANCE_ACCURACY_VALUE',
'Maximum model space distance between geometric entities at asserted c
onnectivities');
#6630=(
GEOMETRIC_REPRESENTATION_CONTEXT(3)
GLOBAL_UNCERTAINTY_ASSIGNED_CONTEXT((#6601))
GLOBAL_UNIT_ASSIGNED_CONTEXT((#6639,#6641,#6642))
REPRESENTATION_CONTEXT('','3D')
);
#6638=(
GEOMETRIC_REPRESENTATION_CONTEXT(3)
GLOBAL_UNCERTAINTY_ASSIGNED_CONTEXT((#6609))
GLOBAL_UNIT_ASSIGNED_CONTEXT((#6639,#6641,#6642))
REPRESENTATION_CONTEXT('','3D')
);
#6639=(
LENGTH_UNIT()
NAMED_UNIT(*)
SI_UNIT(.CENTI.,.METRE.)
);
#6641=(
NAMED_UNIT(*)
PLANE_ANGLE_UNIT()
SI_UNIT($,.RADIAN.)
);
#6642=(
NAMED_UNIT(*)
SI_UNIT($,.STERADIAN.)
SOLID_ANGLE_UNIT()
);
#6663=SHAPE_DEFINITION_REPRESENTATION(#6719,#6757);
#6719=PRODUCT_DEFINITION_SHAPE('',$,#6786);
#6757=SHAPE_REPRESENTATION('',(#4208),#6630);
#6765=PRODUCT_DEFINITION_CONTEXT('part definition',#6851,'design');
#6786=PRODUCT_DEFINITION('Bushing plate','Bushing plate',#6814,#6765);
#6814=PRODUCT_DEFINITION_FORMATION('',$,#6873);
#6851=APPLICATION_CONTEXT(
'Core Data for Automotive Mechanical Design Process');
#6852=PRODUCT_CONTEXT('part definition',#6851,'mechanical');
#6873=PRODUCT('Bushing plate','Bushing plate','Bushing plate',(#6852));
#6951=COLOUR_RGB('Off White',0.89,0.88,0.83);
#6952=FILL_AREA_STYLE_COLOUR('',#6951);
#6953=FILL_AREA_STYLE('',(#6952));
#6954=SURFACE_STYLE_FILL_AREA(#6953);
#6955=SURFACE_SIDE_STYLE('',(#6954));
#6956=SURFACE_STYLE_USAGE(.BOTH.,#6955);
#6957=PRESENTATION_STYLE_ASSIGNMENT((#6956));
ENDSEC;
END-ISO-10303-21;
